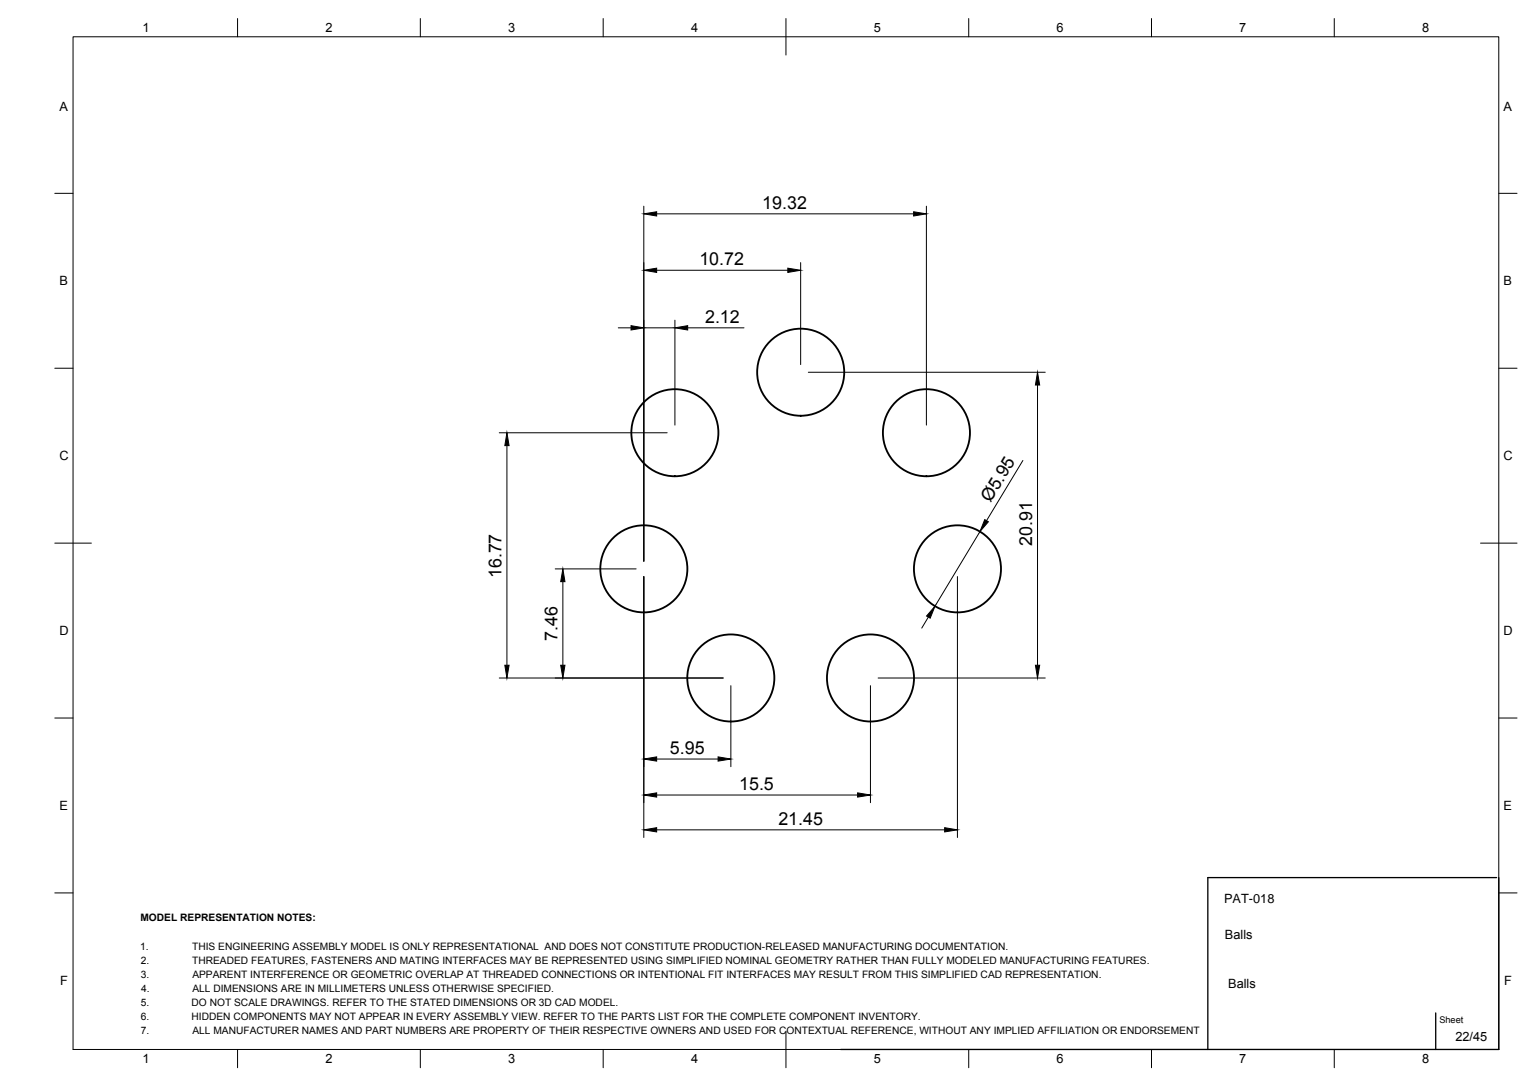
ISO-10303-21;
HEADER;
/* Generated by software containing ST-Developer
 * from STEP Tools, Inc. (www.steptools.com) 
 */

FILE_DESCRIPTION(
/* description */ ('Cam-driven reciprocating slide'),
/* implementation_level */ '2;1');

FILE_NAME(
/* name */ 'Balls.step',
/* time_stamp */ '2026-10-28T03:25:20-07:00',
/* author */ (''),
/* organization */ (''),
/* preprocessor_version */ 'ST-DEVELOPER v20.2',
/* originating_system */ 'Autodesk Translation Framework v15.17.0.0',
/* authorisation */ '');

FILE_SCHEMA (('AUTOMOTIVE_DESIGN { 1 0 10303 214 3 1 1 }'));
ENDSEC;

DATA;
#10=MECHANICAL_DESIGN_GEOMETRIC_PRESENTATION_REPRESENTATION('',(#437,#438,#439,#440,#441,#442,#443),#13277);
#301=SPHERICAL_SURFACE('',#7196,0.29765);
#302=SPHERICAL_SURFACE('',#7198,0.29765);
#303=SPHERICAL_SURFACE('',#7200,0.29765);
#304=SPHERICAL_SURFACE('',#7202,0.29765);
#305=SPHERICAL_SURFACE('',#7204,0.29765);
#306=SPHERICAL_SURFACE('',#7206,0.29765);
#307=SPHERICAL_SURFACE('',#7208,0.29765);
#363=SHAPE_REPRESENTATION_RELATIONSHIP('SRR','None',#13457,#400);
#400=ADVANCED_BREP_SHAPE_REPRESENTATION('',(#481,#482,#483,#484,#485,#486,
#487),#13252);
#437=STYLED_ITEM('',(#13720),#481);
#438=STYLED_ITEM('',(#13720),#482);
#439=STYLED_ITEM('',(#13720),#483);
#440=STYLED_ITEM('',(#13720),#484);
#441=STYLED_ITEM('',(#13720),#485);
#442=STYLED_ITEM('',(#13720),#486);
#443=STYLED_ITEM('',(#13720),#487);
#481=MANIFOLD_SOLID_BREP('Body1',#6413);
#482=MANIFOLD_SOLID_BREP('Body2',#6414);
#483=MANIFOLD_SOLID_BREP('Body3',#6415);
#484=MANIFOLD_SOLID_BREP('Body4',#6416);
#485=MANIFOLD_SOLID_BREP('Body5',#6417);
#486=MANIFOLD_SOLID_BREP('Body6',#6418);
#487=MANIFOLD_SOLID_BREP('Body7',#6419);
#1068=FACE_OUTER_BOUND('',#1562,.T.);
#1069=FACE_OUTER_BOUND('',#1563,.T.);
#1070=FACE_OUTER_BOUND('',#1564,.T.);
#1071=FACE_OUTER_BOUND('',#1565,.T.);
#1072=FACE_OUTER_BOUND('',#1566,.T.);
#1073=FACE_OUTER_BOUND('',#1567,.T.);
#1074=FACE_OUTER_BOUND('',#1568,.T.);
#1562=EDGE_LOOP('',(#5072,#5073));
#1563=EDGE_LOOP('',(#5074,#5075));
#1564=EDGE_LOOP('',(#5076,#5077));
#1565=EDGE_LOOP('',(#5078,#5079));
#1566=EDGE_LOOP('',(#5080,#5081));
#1567=EDGE_LOOP('',(#5082,#5083));
#1568=EDGE_LOOP('',(#5084,#5085));
#2869=CIRCLE('',#7197,0.29765);
#2870=CIRCLE('',#7199,0.29765);
#2871=CIRCLE('',#7201,0.29765);
#2872=CIRCLE('',#7203,0.29765);
#2873=CIRCLE('',#7205,0.29765);
#2874=CIRCLE('',#7207,0.29765);
#2875=CIRCLE('',#7209,0.29765);
#3279=VERTEX_POINT('',#11901);
#3280=VERTEX_POINT('',#11902);
#3281=VERTEX_POINT('',#11905);
#3282=VERTEX_POINT('',#11906);
#3283=VERTEX_POINT('',#11909);
#3284=VERTEX_POINT('',#11910);
#3285=VERTEX_POINT('',#11913);
#3286=VERTEX_POINT('',#11914);
#3287=VERTEX_POINT('',#11917);
#3288=VERTEX_POINT('',#11918);
#3289=VERTEX_POINT('',#11921);
#3290=VERTEX_POINT('',#11922);
#3291=VERTEX_POINT('',#11925);
#3292=VERTEX_POINT('',#11926);
#3926=EDGE_CURVE('',#3279,#3280,#2869,.T.);
#3927=EDGE_CURVE('',#3281,#3282,#2870,.T.);
#3928=EDGE_CURVE('',#3283,#3284,#2871,.T.);
#3929=EDGE_CURVE('',#3285,#3286,#2872,.T.);
#3930=EDGE_CURVE('',#3287,#3288,#2873,.T.);
#3931=EDGE_CURVE('',#3289,#3290,#2874,.T.);
#3932=EDGE_CURVE('',#3291,#3292,#2875,.T.);
#5072=ORIENTED_EDGE('',*,*,#3926,.T.);
#5073=ORIENTED_EDGE('',*,*,#3926,.F.);
#5074=ORIENTED_EDGE('',*,*,#3927,.T.);
#5075=ORIENTED_EDGE('',*,*,#3927,.F.);
#5076=ORIENTED_EDGE('',*,*,#3928,.T.);
#5077=ORIENTED_EDGE('',*,*,#3928,.F.);
#5078=ORIENTED_EDGE('',*,*,#3929,.T.);
#5079=ORIENTED_EDGE('',*,*,#3929,.F.);
#5080=ORIENTED_EDGE('',*,*,#3930,.T.);
#5081=ORIENTED_EDGE('',*,*,#3930,.F.);
#5082=ORIENTED_EDGE('',*,*,#3931,.T.);
#5083=ORIENTED_EDGE('',*,*,#3931,.F.);
#5084=ORIENTED_EDGE('',*,*,#3932,.T.);
#5085=ORIENTED_EDGE('',*,*,#3932,.F.);
#6186=ADVANCED_FACE('',(#1068),#301,.T.);
#6187=ADVANCED_FACE('',(#1069),#302,.T.);
#6188=ADVANCED_FACE('',(#1070),#303,.T.);
#6189=ADVANCED_FACE('',(#1071),#304,.T.);
#6190=ADVANCED_FACE('',(#1072),#305,.T.);
#6191=ADVANCED_FACE('',(#1073),#306,.T.);
#6192=ADVANCED_FACE('',(#1074),#307,.T.);
#6413=CLOSED_SHELL('',(#6186));
#6414=CLOSED_SHELL('',(#6187));
#6415=CLOSED_SHELL('',(#6188));
#6416=CLOSED_SHELL('',(#6189));
#6417=CLOSED_SHELL('',(#6190));
#6418=CLOSED_SHELL('',(#6191));
#6419=CLOSED_SHELL('',(#6192));
#7195=AXIS2_PLACEMENT_3D('',#11899,#8562,#8563);
#7196=AXIS2_PLACEMENT_3D('',#11900,#8564,#8565);
#7197=AXIS2_PLACEMENT_3D('',#11903,#8566,#8567);
#7198=AXIS2_PLACEMENT_3D('',#11904,#8568,#8569);
#7199=AXIS2_PLACEMENT_3D('',#11907,#8570,#8571);
#7200=AXIS2_PLACEMENT_3D('',#11908,#8572,#8573);
#7201=AXIS2_PLACEMENT_3D('',#11911,#8574,#8575);
#7202=AXIS2_PLACEMENT_3D('',#11912,#8576,#8577);
#7203=AXIS2_PLACEMENT_3D('',#11915,#8578,#8579);
#7204=AXIS2_PLACEMENT_3D('',#11916,#8580,#8581);
#7205=AXIS2_PLACEMENT_3D('',#11919,#8582,#8583);
#7206=AXIS2_PLACEMENT_3D('',#11920,#8584,#8585);
#7207=AXIS2_PLACEMENT_3D('',#11923,#8586,#8587);
#7208=AXIS2_PLACEMENT_3D('',#11924,#8588,#8589);
#7209=AXIS2_PLACEMENT_3D('',#11927,#8590,#8591);
#8562=DIRECTION('axis',(0.,0.,1.));
#8563=DIRECTION('refdir',(1.,0.,0.));
#8564=DIRECTION('center_axis',(0.,0.,1.));
#8565=DIRECTION('ref_axis',(1.,0.,0.));
#8566=DIRECTION('center_axis',(1.22464679914735E-16,-1.,0.));
#8567=DIRECTION('ref_axis',(-1.,-1.22464679914735E-16,0.));
#8568=DIRECTION('center_axis',(0.78183148246803,0.,0.623489801858733));
#8569=DIRECTION('ref_axis',(0.623489801858734,0.,-0.78183148246803));
#8570=DIRECTION('center_axis',(7.63554790147315E-17,-1.,-9.57467422477103E-17));
#8571=DIRECTION('ref_axis',(-0.623489801858734,-1.22464679914735E-16,0.78183148246803));
#8572=DIRECTION('center_axis',(0.974927912181824,0.,-0.222520933956314));
#8573=DIRECTION('ref_axis',(-0.222520933956314,0.,-0.974927912181824));
#8574=DIRECTION('center_axis',(-2.7250954951288E-17,-1.,-1.19394234705288E-16));
#8575=DIRECTION('ref_axis',(0.222520933956314,-1.22464679914735E-16,0.974927912181824));
#8576=DIRECTION('center_axis',(0.433883739117558,0.,-0.900968867902419));
#8577=DIRECTION('ref_axis',(-0.900968867902419,0.,-0.433883739117558));
#8578=DIRECTION('center_axis',(-1.10336864020811E-16,-1.,-5.31354332312403E-17));
#8579=DIRECTION('ref_axis',(0.900968867902419,-1.22464679914735E-16,0.433883739117558));
#8580=DIRECTION('center_axis',(-0.433883739117558,0.,-0.900968867902419));
#8581=DIRECTION('ref_axis',(-0.900968867902419,0.,0.433883739117558));
#8582=DIRECTION('center_axis',(-1.10336864020811E-16,-1.,5.31354332312403E-17));
#8583=DIRECTION('ref_axis',(0.900968867902419,-1.22464679914735E-16,-0.433883739117558));
#8584=DIRECTION('center_axis',(-0.974927912181824,0.,-0.222520933956314));
#8585=DIRECTION('ref_axis',(-0.222520933956315,0.,0.974927912181824));
#8586=DIRECTION('center_axis',(-2.7250954951288E-17,-1.,1.19394234705288E-16));
#8587=DIRECTION('ref_axis',(0.222520933956315,-1.22464679914735E-16,-0.974927912181824));
#8588=DIRECTION('center_axis',(-0.78183148246803,0.,0.623489801858734));
#8589=DIRECTION('ref_axis',(0.623489801858733,0.,0.78183148246803));
#8590=DIRECTION('center_axis',(7.63554790147315E-17,-1.,9.57467422477103E-17));
#8591=DIRECTION('ref_axis',(-0.623489801858733,-1.22464679914735E-16,-0.78183148246803));
#11899=CARTESIAN_POINT('',(0.,0.,0.));
#11900=CARTESIAN_POINT('Origin',(1.1,0.,0.));
#11901=CARTESIAN_POINT('',(1.1,-2.23201749654651E-33,0.29765));
#11902=CARTESIAN_POINT('',(1.1,-2.23201749654651E-33,-0.29765));
#11903=CARTESIAN_POINT('Origin',(1.1,0.,0.));
#11904=CARTESIAN_POINT('Origin',(0.685838782044607,0.,-0.860014630714833));
#11905=CARTESIAN_POINT('',(0.918550922801216,-5.31350540756609E-33,-0.674432891191581));
#11906=CARTESIAN_POINT('',(0.453126641287998,8.49470414473068E-34,-1.04559637023808));
#11907=CARTESIAN_POINT('Origin',(0.685838782044607,0.,-0.860014630714833));
#11908=CARTESIAN_POINT('Origin',(-0.244773027351946,0.,-1.07242070340001));
#11909=CARTESIAN_POINT('',(0.0454142657089739,-2.23201749654651E-33,-1.1386540593921));
#11910=CARTESIAN_POINT('',(-0.534960320412865,-2.23201749654651E-33,-1.00618734740791));
#11911=CARTESIAN_POINT('Origin',(-0.244773027351946,0.,-1.07242070340001));
#11912=CARTESIAN_POINT('Origin',(-0.991065754692661,0.,-0.477272113029314));
#11913=CARTESIAN_POINT('',(-0.86192025974432,8.49470414473067E-34,-0.745445496560469));
#11914=CARTESIAN_POINT('',(-1.120211249641,-5.31350540756609E-33,-0.209098729498159));
#11915=CARTESIAN_POINT('Origin',(-0.991065754692661,0.,-0.477272113029314));
#11916=CARTESIAN_POINT('Origin',(-0.991065754692661,0.,0.477272113029314));
#11917=CARTESIAN_POINT('',(-1.120211249641,-2.23201749654651E-33,0.209098729498159));
#11918=CARTESIAN_POINT('',(-0.86192025974432,-2.23201749654651E-33,0.745445496560469));
#11919=CARTESIAN_POINT('Origin',(-0.991065754692661,0.,0.477272113029314));
#11920=CARTESIAN_POINT('Origin',(-0.244773027351946,0.,1.07242070340001));
#11921=CARTESIAN_POINT('',(-0.534960320412866,-2.23201749654651E-33,1.00618734740791));
#11922=CARTESIAN_POINT('',(0.0454142657089737,-2.23201749654651E-33,1.1386540593921));
#11923=CARTESIAN_POINT('Origin',(-0.244773027351946,0.,1.07242070340001));
#11924=CARTESIAN_POINT('Origin',(0.685838782044607,0.,0.860014630714833));
#11925=CARTESIAN_POINT('',(0.453126641287998,-2.23201749654651E-33,1.04559637023808));
#11926=CARTESIAN_POINT('',(0.918550922801216,-2.23201749654651E-33,0.674432891191581));
#11927=CARTESIAN_POINT('Origin',(0.685838782044607,0.,0.860014630714833));
#13208=UNCERTAINTY_MEASURE_WITH_UNIT(LENGTH_MEASURE(0.001),#13278,
'DISTANCE_ACCURACY_VALUE',
'Maximum model space distance between geometric entities at asserted c
onnectivities');
#13233=UNCERTAINTY_MEASURE_WITH_UNIT(LENGTH_MEASURE(0.001),#13278,
'DISTANCE_ACCURACY_VALUE',
'Maximum model space distance between geometric entities at asserted c
onnectivities');
#13252=(
GEOMETRIC_REPRESENTATION_CONTEXT(3)
GLOBAL_UNCERTAINTY_ASSIGNED_CONTEXT((#13208))
GLOBAL_UNIT_ASSIGNED_CONTEXT((#13278,#13280,#13281))
REPRESENTATION_CONTEXT('','3D')
);
#13277=(
GEOMETRIC_REPRESENTATION_CONTEXT(3)
GLOBAL_UNCERTAINTY_ASSIGNED_CONTEXT((#13233))
GLOBAL_UNIT_ASSIGNED_CONTEXT((#13278,#13280,#13281))
REPRESENTATION_CONTEXT('','3D')
);
#13278=(
LENGTH_UNIT()
NAMED_UNIT(*)
SI_UNIT(.CENTI.,.METRE.)
);
#13280=(
NAMED_UNIT(*)
PLANE_ANGLE_UNIT()
SI_UNIT($,.RADIAN.)
);
#13281=(
NAMED_UNIT(*)
SI_UNIT($,.STERADIAN.)
SOLID_ANGLE_UNIT()
);
#13300=SHAPE_DEFINITION_REPRESENTATION(#13343,#13457);
#13343=PRODUCT_DEFINITION_SHAPE('',$,#13501);
#13457=SHAPE_REPRESENTATION('',(#7195),#13252);
#13482=PRODUCT_DEFINITION_CONTEXT('part definition',#13613,'design');
#13501=PRODUCT_DEFINITION('Balls','Balls',#13544,#13482);
#13544=PRODUCT_DEFINITION_FORMATION('',$,#13633);
#13613=APPLICATION_CONTEXT(
'Core Data for Automotive Mechanical Design Process');
#13614=PRODUCT_CONTEXT('part definition',#13613,'mechanical');
#13633=PRODUCT('Balls','Balls','Balls',(#13614));
#13714=COLOUR_RGB('Grey',0.48,0.52,0.57);
#13715=FILL_AREA_STYLE_COLOUR('',#13714);
#13716=FILL_AREA_STYLE('',(#13715));
#13717=SURFACE_STYLE_FILL_AREA(#13716);
#13718=SURFACE_SIDE_STYLE('',(#13717));
#13719=SURFACE_STYLE_USAGE(.BOTH.,#13718);
#13720=PRESENTATION_STYLE_ASSIGNMENT((#13719));
ENDSEC;
END-ISO-10303-21;
